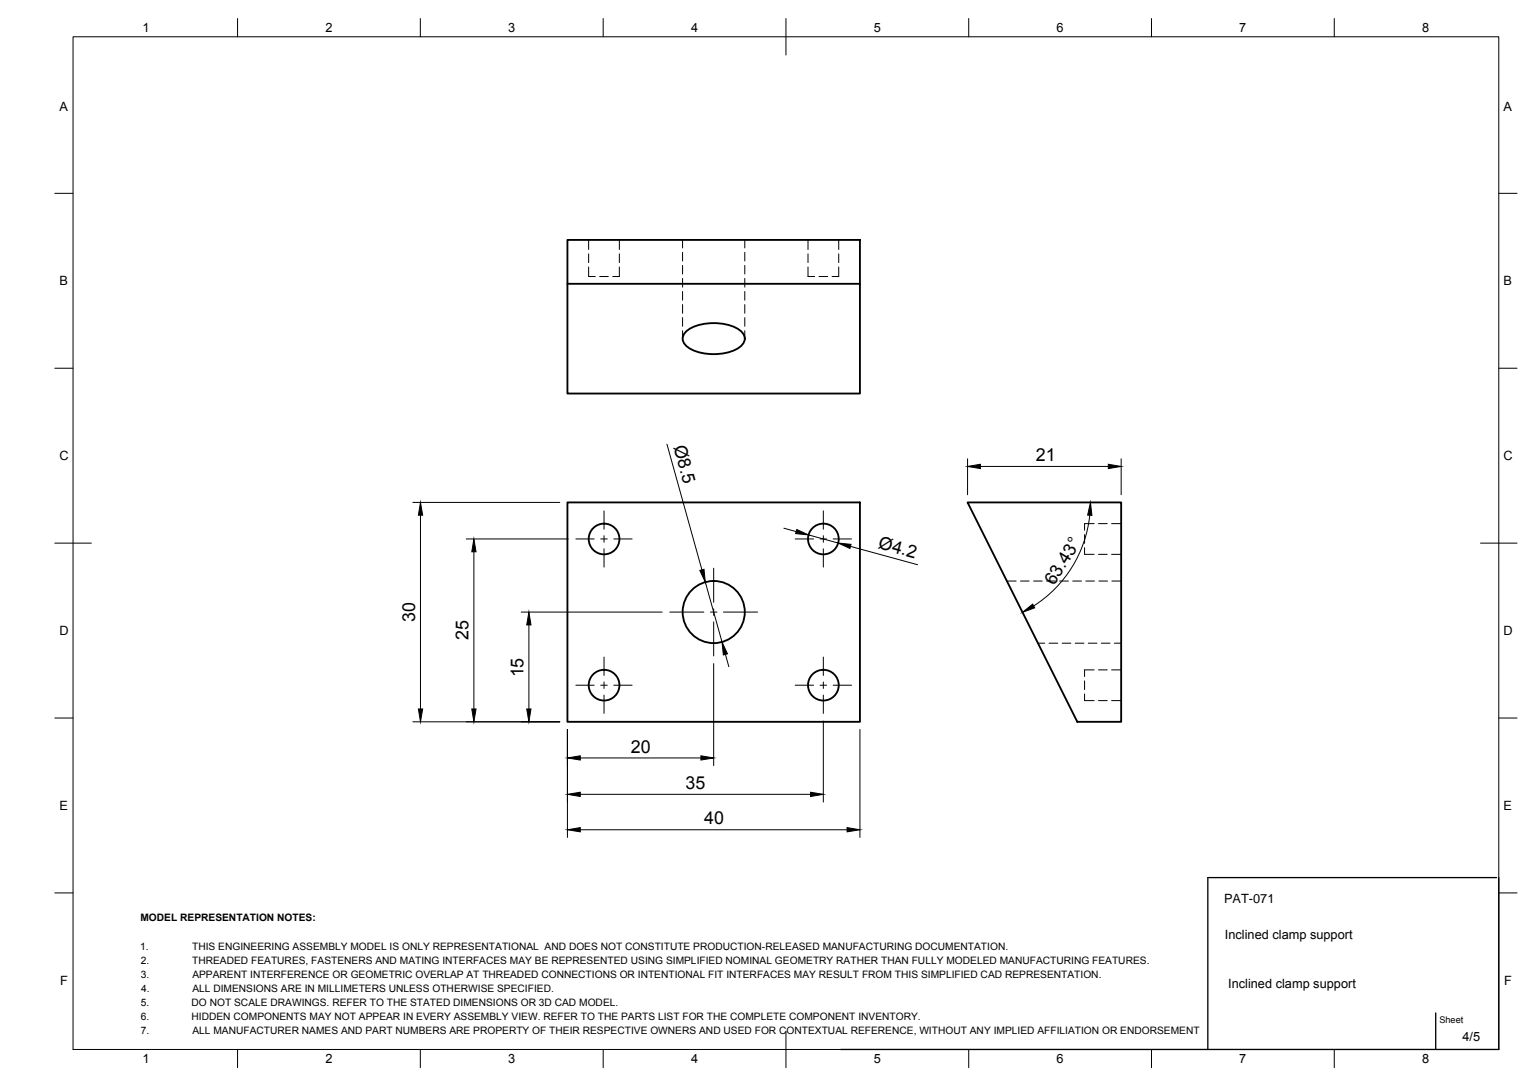
ISO-10303-21;
HEADER;
/* Generated by software containing ST-Developer
 * from STEP Tools, Inc. (www.steptools.com) 
 */

FILE_DESCRIPTION(
/* description */ ('Low-profile wedge edge clamp'),
/* implementation_level */ '2;1');

FILE_NAME(
/* name */ 'Inclined clamp support.step',
/* time_stamp */ '2026-10-29T15:58:13-07:00',
/* author */ (''),
/* organization */ (''),
/* preprocessor_version */ 'ST-DEVELOPER v20.2',
/* originating_system */ 'Autodesk Translation Framework v15.17.0.0',
/* authorisation */ '');

FILE_SCHEMA (('AUTOMOTIVE_DESIGN { 1 0 10303 214 3 1 1 }'));
ENDSEC;

DATA;
#10=MECHANICAL_DESIGN_GEOMETRIC_PRESENTATION_REPRESENTATION('',(#80),#2996);
#64=ELLIPSE('',#1900,0.475164445218705,0.425);
#68=SHAPE_REPRESENTATION_RELATIONSHIP('SRR','None',#3030,#74);
#74=ADVANCED_BREP_SHAPE_REPRESENTATION('',(#86),#2991);
#80=STYLED_ITEM('',(#3119),#86);
#86=MANIFOLD_SOLID_BREP('Body1',#1709);
#150=FACE_BOUND('',#408,.T.);
#151=FACE_BOUND('',#409,.T.);
#152=FACE_BOUND('',#410,.T.);
#153=FACE_BOUND('',#411,.T.);
#154=FACE_BOUND('',#412,.T.);
#155=FACE_BOUND('',#415,.T.);
#168=PLANE('',#1885);
#169=PLANE('',#1889);
#170=PLANE('',#1893);
#171=PLANE('',#1897);
#172=PLANE('',#1901);
#173=PLANE('',#1902);
#174=PLANE('',#1903);
#175=PLANE('',#1904);
#176=PLANE('',#1905);
#177=PLANE('',#1906);
#244=FACE_OUTER_BOUND('',#397,.T.);
#245=FACE_OUTER_BOUND('',#398,.T.);
#246=FACE_OUTER_BOUND('',#399,.T.);
#247=FACE_OUTER_BOUND('',#400,.T.);
#248=FACE_OUTER_BOUND('',#401,.T.);
#249=FACE_OUTER_BOUND('',#402,.T.);
#250=FACE_OUTER_BOUND('',#403,.T.);
#251=FACE_OUTER_BOUND('',#404,.T.);
#252=FACE_OUTER_BOUND('',#405,.T.);
#253=FACE_OUTER_BOUND('',#406,.T.);
#254=FACE_OUTER_BOUND('',#407,.T.);
#255=FACE_OUTER_BOUND('',#413,.T.);
#256=FACE_OUTER_BOUND('',#414,.T.);
#257=FACE_OUTER_BOUND('',#416,.T.);
#258=FACE_OUTER_BOUND('',#417,.T.);
#397=EDGE_LOOP('',(#1349,#1350,#1351,#1352));
#398=EDGE_LOOP('',(#1353));
#399=EDGE_LOOP('',(#1354,#1355,#1356,#1357));
#400=EDGE_LOOP('',(#1358));
#401=EDGE_LOOP('',(#1359,#1360,#1361,#1362));
#402=EDGE_LOOP('',(#1363));
#403=EDGE_LOOP('',(#1364,#1365,#1366,#1367));
#404=EDGE_LOOP('',(#1368));
#405=EDGE_LOOP('',(#1369,#1370,#1371,#1372));
#406=EDGE_LOOP('',(#1373,#1374,#1375,#1376));
#407=EDGE_LOOP('',(#1377,#1378,#1379,#1380));
#408=EDGE_LOOP('',(#1381));
#409=EDGE_LOOP('',(#1382));
#410=EDGE_LOOP('',(#1383));
#411=EDGE_LOOP('',(#1384));
#412=EDGE_LOOP('',(#1385));
#413=EDGE_LOOP('',(#1386,#1387,#1388,#1389));
#414=EDGE_LOOP('',(#1390,#1391,#1392,#1393));
#415=EDGE_LOOP('',(#1394));
#416=EDGE_LOOP('',(#1395,#1396,#1397,#1398));
#417=EDGE_LOOP('',(#1399,#1400,#1401,#1402));
#508=LINE('',#2715,#627);
#509=LINE('',#2722,#628);
#510=LINE('',#2729,#629);
#511=LINE('',#2736,#630);
#512=LINE('',#2743,#631);
#513=LINE('',#2748,#632);
#514=LINE('',#2750,#633);
#515=LINE('',#2752,#634);
#516=LINE('',#2753,#635);
#517=LINE('',#2756,#636);
#518=LINE('',#2758,#637);
#519=LINE('',#2759,#638);
#520=LINE('',#2762,#639);
#521=LINE('',#2764,#640);
#522=LINE('',#2765,#641);
#523=LINE('',#2767,#642);
#524=LINE('',#2768,#643);
#627=VECTOR('',#2228,0.21);
#628=VECTOR('',#2237,0.21);
#629=VECTOR('',#2246,0.21);
#630=VECTOR('',#2255,0.21);
#631=VECTOR('',#2264,0.425);
#632=VECTOR('',#2269,1.);
#633=VECTOR('',#2270,1.);
#634=VECTOR('',#2271,1.);
#635=VECTOR('',#2272,1.);
#636=VECTOR('',#2275,1.);
#637=VECTOR('',#2276,1.);
#638=VECTOR('',#2277,1.);
#639=VECTOR('',#2280,1.);
#640=VECTOR('',#2281,1.);
#641=VECTOR('',#2282,1.);
#642=VECTOR('',#2285,1.);
#643=VECTOR('',#2286,1.);
#764=CIRCLE('',#1883,0.21);
#765=CIRCLE('',#1884,0.21);
#766=CIRCLE('',#1887,0.21);
#767=CIRCLE('',#1888,0.21);
#768=CIRCLE('',#1891,0.21);
#769=CIRCLE('',#1892,0.21);
#770=CIRCLE('',#1895,0.21);
#771=CIRCLE('',#1896,0.21);
#772=CIRCLE('',#1899,0.425);
#858=VERTEX_POINT('',#2712);
#859=VERTEX_POINT('',#2714);
#860=VERTEX_POINT('',#2719);
#861=VERTEX_POINT('',#2721);
#862=VERTEX_POINT('',#2726);
#863=VERTEX_POINT('',#2728);
#864=VERTEX_POINT('',#2733);
#865=VERTEX_POINT('',#2735);
#866=VERTEX_POINT('',#2740);
#867=VERTEX_POINT('',#2742);
#868=VERTEX_POINT('',#2746);
#869=VERTEX_POINT('',#2747);
#870=VERTEX_POINT('',#2749);
#871=VERTEX_POINT('',#2751);
#872=VERTEX_POINT('',#2755);
#873=VERTEX_POINT('',#2757);
#874=VERTEX_POINT('',#2761);
#875=VERTEX_POINT('',#2763);
#1033=EDGE_CURVE('',#858,#858,#764,.T.);
#1034=EDGE_CURVE('',#858,#859,#508,.T.);
#1035=EDGE_CURVE('',#859,#859,#765,.T.);
#1036=EDGE_CURVE('',#860,#860,#766,.T.);
#1037=EDGE_CURVE('',#860,#861,#509,.T.);
#1038=EDGE_CURVE('',#861,#861,#767,.T.);
#1039=EDGE_CURVE('',#862,#862,#768,.T.);
#1040=EDGE_CURVE('',#862,#863,#510,.T.);
#1041=EDGE_CURVE('',#863,#863,#769,.T.);
#1042=EDGE_CURVE('',#864,#864,#770,.T.);
#1043=EDGE_CURVE('',#864,#865,#511,.T.);
#1044=EDGE_CURVE('',#865,#865,#771,.T.);
#1045=EDGE_CURVE('',#866,#866,#772,.T.);
#1046=EDGE_CURVE('',#866,#867,#512,.T.);
#1047=EDGE_CURVE('',#867,#867,#64,.T.);
#1048=EDGE_CURVE('',#868,#869,#513,.T.);
#1049=EDGE_CURVE('',#868,#870,#514,.T.);
#1050=EDGE_CURVE('',#871,#870,#515,.T.);
#1051=EDGE_CURVE('',#869,#871,#516,.T.);
#1052=EDGE_CURVE('',#869,#872,#517,.T.);
#1053=EDGE_CURVE('',#873,#871,#518,.T.);
#1054=EDGE_CURVE('',#872,#873,#519,.T.);
#1055=EDGE_CURVE('',#872,#874,#520,.T.);
#1056=EDGE_CURVE('',#875,#873,#521,.T.);
#1057=EDGE_CURVE('',#874,#875,#522,.T.);
#1058=EDGE_CURVE('',#874,#868,#523,.T.);
#1059=EDGE_CURVE('',#870,#875,#524,.T.);
#1349=ORIENTED_EDGE('',*,*,#1033,.F.);
#1350=ORIENTED_EDGE('',*,*,#1034,.T.);
#1351=ORIENTED_EDGE('',*,*,#1035,.T.);
#1352=ORIENTED_EDGE('',*,*,#1034,.F.);
#1353=ORIENTED_EDGE('',*,*,#1035,.F.);
#1354=ORIENTED_EDGE('',*,*,#1036,.F.);
#1355=ORIENTED_EDGE('',*,*,#1037,.T.);
#1356=ORIENTED_EDGE('',*,*,#1038,.T.);
#1357=ORIENTED_EDGE('',*,*,#1037,.F.);
#1358=ORIENTED_EDGE('',*,*,#1038,.F.);
#1359=ORIENTED_EDGE('',*,*,#1039,.F.);
#1360=ORIENTED_EDGE('',*,*,#1040,.T.);
#1361=ORIENTED_EDGE('',*,*,#1041,.T.);
#1362=ORIENTED_EDGE('',*,*,#1040,.F.);
#1363=ORIENTED_EDGE('',*,*,#1041,.F.);
#1364=ORIENTED_EDGE('',*,*,#1042,.F.);
#1365=ORIENTED_EDGE('',*,*,#1043,.T.);
#1366=ORIENTED_EDGE('',*,*,#1044,.T.);
#1367=ORIENTED_EDGE('',*,*,#1043,.F.);
#1368=ORIENTED_EDGE('',*,*,#1044,.F.);
#1369=ORIENTED_EDGE('',*,*,#1045,.F.);
#1370=ORIENTED_EDGE('',*,*,#1046,.T.);
#1371=ORIENTED_EDGE('',*,*,#1047,.F.);
#1372=ORIENTED_EDGE('',*,*,#1046,.F.);
#1373=ORIENTED_EDGE('',*,*,#1048,.F.);
#1374=ORIENTED_EDGE('',*,*,#1049,.T.);
#1375=ORIENTED_EDGE('',*,*,#1050,.F.);
#1376=ORIENTED_EDGE('',*,*,#1051,.F.);
#1377=ORIENTED_EDGE('',*,*,#1052,.F.);
#1378=ORIENTED_EDGE('',*,*,#1051,.T.);
#1379=ORIENTED_EDGE('',*,*,#1053,.F.);
#1380=ORIENTED_EDGE('',*,*,#1054,.F.);
#1381=ORIENTED_EDGE('',*,*,#1045,.T.);
#1382=ORIENTED_EDGE('',*,*,#1042,.T.);
#1383=ORIENTED_EDGE('',*,*,#1039,.T.);
#1384=ORIENTED_EDGE('',*,*,#1036,.T.);
#1385=ORIENTED_EDGE('',*,*,#1033,.T.);
#1386=ORIENTED_EDGE('',*,*,#1055,.F.);
#1387=ORIENTED_EDGE('',*,*,#1054,.T.);
#1388=ORIENTED_EDGE('',*,*,#1056,.F.);
#1389=ORIENTED_EDGE('',*,*,#1057,.F.);
#1390=ORIENTED_EDGE('',*,*,#1058,.F.);
#1391=ORIENTED_EDGE('',*,*,#1057,.T.);
#1392=ORIENTED_EDGE('',*,*,#1059,.F.);
#1393=ORIENTED_EDGE('',*,*,#1049,.F.);
#1394=ORIENTED_EDGE('',*,*,#1047,.T.);
#1395=ORIENTED_EDGE('',*,*,#1059,.T.);
#1396=ORIENTED_EDGE('',*,*,#1056,.T.);
#1397=ORIENTED_EDGE('',*,*,#1053,.T.);
#1398=ORIENTED_EDGE('',*,*,#1050,.T.);
#1399=ORIENTED_EDGE('',*,*,#1058,.T.);
#1400=ORIENTED_EDGE('',*,*,#1048,.T.);
#1401=ORIENTED_EDGE('',*,*,#1052,.T.);
#1402=ORIENTED_EDGE('',*,*,#1055,.T.);
#1603=CYLINDRICAL_SURFACE('',#1882,0.21);
#1604=CYLINDRICAL_SURFACE('',#1886,0.21);
#1605=CYLINDRICAL_SURFACE('',#1890,0.21);
#1606=CYLINDRICAL_SURFACE('',#1894,0.21);
#1607=CYLINDRICAL_SURFACE('',#1898,0.425);
#1651=ADVANCED_FACE('',(#244),#1603,.F.);
#1652=ADVANCED_FACE('',(#245),#168,.F.);
#1653=ADVANCED_FACE('',(#246),#1604,.F.);
#1654=ADVANCED_FACE('',(#247),#169,.F.);
#1655=ADVANCED_FACE('',(#248),#1605,.F.);
#1656=ADVANCED_FACE('',(#249),#170,.F.);
#1657=ADVANCED_FACE('',(#250),#1606,.F.);
#1658=ADVANCED_FACE('',(#251),#171,.F.);
#1659=ADVANCED_FACE('',(#252),#1607,.F.);
#1660=ADVANCED_FACE('',(#253),#172,.T.);
#1661=ADVANCED_FACE('',(#254,#150,#151,#152,#153,#154),#173,.T.);
#1662=ADVANCED_FACE('',(#255),#174,.T.);
#1663=ADVANCED_FACE('',(#256,#155),#175,.T.);
#1664=ADVANCED_FACE('',(#257),#176,.T.);
#1665=ADVANCED_FACE('',(#258),#177,.F.);
#1709=CLOSED_SHELL('',(#1651,#1652,#1653,#1654,#1655,#1656,#1657,#1658,
#1659,#1660,#1661,#1662,#1663,#1664,#1665));
#1881=AXIS2_PLACEMENT_3D('',#2710,#2222,#2223);
#1882=AXIS2_PLACEMENT_3D('',#2711,#2224,#2225);
#1883=AXIS2_PLACEMENT_3D('',#2713,#2226,#2227);
#1884=AXIS2_PLACEMENT_3D('',#2716,#2229,#2230);
#1885=AXIS2_PLACEMENT_3D('',#2717,#2231,#2232);
#1886=AXIS2_PLACEMENT_3D('',#2718,#2233,#2234);
#1887=AXIS2_PLACEMENT_3D('',#2720,#2235,#2236);
#1888=AXIS2_PLACEMENT_3D('',#2723,#2238,#2239);
#1889=AXIS2_PLACEMENT_3D('',#2724,#2240,#2241);
#1890=AXIS2_PLACEMENT_3D('',#2725,#2242,#2243);
#1891=AXIS2_PLACEMENT_3D('',#2727,#2244,#2245);
#1892=AXIS2_PLACEMENT_3D('',#2730,#2247,#2248);
#1893=AXIS2_PLACEMENT_3D('',#2731,#2249,#2250);
#1894=AXIS2_PLACEMENT_3D('',#2732,#2251,#2252);
#1895=AXIS2_PLACEMENT_3D('',#2734,#2253,#2254);
#1896=AXIS2_PLACEMENT_3D('',#2737,#2256,#2257);
#1897=AXIS2_PLACEMENT_3D('',#2738,#2258,#2259);
#1898=AXIS2_PLACEMENT_3D('',#2739,#2260,#2261);
#1899=AXIS2_PLACEMENT_3D('',#2741,#2262,#2263);
#1900=AXIS2_PLACEMENT_3D('',#2744,#2265,#2266);
#1901=AXIS2_PLACEMENT_3D('',#2745,#2267,#2268);
#1902=AXIS2_PLACEMENT_3D('',#2754,#2273,#2274);
#1903=AXIS2_PLACEMENT_3D('',#2760,#2278,#2279);
#1904=AXIS2_PLACEMENT_3D('',#2766,#2283,#2284);
#1905=AXIS2_PLACEMENT_3D('',#2769,#2287,#2288);
#1906=AXIS2_PLACEMENT_3D('',#2770,#2289,#2290);
#2222=DIRECTION('axis',(0.,0.,1.));
#2223=DIRECTION('refdir',(1.,0.,0.));
#2224=DIRECTION('center_axis',(0.,0.,1.));
#2225=DIRECTION('ref_axis',(1.,0.,0.));
#2226=DIRECTION('center_axis',(0.,0.,1.));
#2227=DIRECTION('ref_axis',(1.,0.,0.));
#2228=DIRECTION('',(0.,0.,1.));
#2229=DIRECTION('center_axis',(0.,0.,1.));
#2230=DIRECTION('ref_axis',(1.,0.,0.));
#2231=DIRECTION('center_axis',(0.,0.,1.));
#2232=DIRECTION('ref_axis',(1.,0.,0.));
#2233=DIRECTION('center_axis',(0.,0.,1.));
#2234=DIRECTION('ref_axis',(1.,0.,0.));
#2235=DIRECTION('center_axis',(0.,0.,1.));
#2236=DIRECTION('ref_axis',(1.,0.,0.));
#2237=DIRECTION('',(0.,0.,1.));
#2238=DIRECTION('center_axis',(0.,0.,1.));
#2239=DIRECTION('ref_axis',(1.,0.,0.));
#2240=DIRECTION('center_axis',(0.,0.,1.));
#2241=DIRECTION('ref_axis',(1.,0.,0.));
#2242=DIRECTION('center_axis',(0.,0.,1.));
#2243=DIRECTION('ref_axis',(1.,0.,0.));
#2244=DIRECTION('center_axis',(0.,0.,1.));
#2245=DIRECTION('ref_axis',(1.,0.,0.));
#2246=DIRECTION('',(0.,0.,1.));
#2247=DIRECTION('center_axis',(0.,0.,1.));
#2248=DIRECTION('ref_axis',(1.,0.,0.));
#2249=DIRECTION('center_axis',(0.,0.,1.));
#2250=DIRECTION('ref_axis',(1.,0.,0.));
#2251=DIRECTION('center_axis',(0.,0.,1.));
#2252=DIRECTION('ref_axis',(1.,0.,0.));
#2253=DIRECTION('center_axis',(0.,0.,1.));
#2254=DIRECTION('ref_axis',(1.,0.,0.));
#2255=DIRECTION('',(0.,0.,1.));
#2256=DIRECTION('center_axis',(0.,0.,1.));
#2257=DIRECTION('ref_axis',(1.,0.,0.));
#2258=DIRECTION('center_axis',(0.,0.,1.));
#2259=DIRECTION('ref_axis',(1.,0.,0.));
#2260=DIRECTION('center_axis',(0.,0.,1.));
#2261=DIRECTION('ref_axis',(1.,0.,0.));
#2262=DIRECTION('center_axis',(0.,0.,1.));
#2263=DIRECTION('ref_axis',(1.,0.,0.));
#2264=DIRECTION('',(0.,0.,1.));
#2265=DIRECTION('center_axis',(0.447213595499958,0.,-0.894427190999916));
#2266=DIRECTION('ref_axis',(0.894427190999916,0.,0.447213595499958));
#2267=DIRECTION('center_axis',(-1.,0.,0.));
#2268=DIRECTION('ref_axis',(0.,0.,1.));
#2269=DIRECTION('',(0.,0.,-1.));
#2270=DIRECTION('',(0.,1.,0.));
#2271=DIRECTION('',(0.,0.,1.));
#2272=DIRECTION('',(0.,1.,0.));
#2273=DIRECTION('center_axis',(0.,0.,-1.));
#2274=DIRECTION('ref_axis',(-1.,0.,0.));
#2275=DIRECTION('',(1.,0.,0.));
#2276=DIRECTION('',(-1.,0.,0.));
#2277=DIRECTION('',(0.,1.,0.));
#2278=DIRECTION('center_axis',(1.,0.,0.));
#2279=DIRECTION('ref_axis',(0.,0.,-1.));
#2280=DIRECTION('',(0.,0.,1.));
#2281=DIRECTION('',(0.,0.,-1.));
#2282=DIRECTION('',(0.,1.,0.));
#2283=DIRECTION('center_axis',(-0.447213595499958,0.,0.894427190999916));
#2284=DIRECTION('ref_axis',(0.894427190999916,0.,0.447213595499958));
#2285=DIRECTION('',(-0.894427190999916,0.,-0.447213595499958));
#2286=DIRECTION('',(0.894427190999916,0.,0.447213595499958));
#2287=DIRECTION('center_axis',(0.,1.,0.));
#2288=DIRECTION('ref_axis',(0.,0.,1.));
#2289=DIRECTION('center_axis',(0.,1.,0.));
#2290=DIRECTION('ref_axis',(1.,0.,0.));
#2710=CARTESIAN_POINT('',(0.,0.,0.));
#2711=CARTESIAN_POINT('Origin',(2.5,-1.5,0.9));
#2712=CARTESIAN_POINT('',(2.29,-1.5,1.));
#2713=CARTESIAN_POINT('Origin',(2.5,-1.5,1.));
#2714=CARTESIAN_POINT('',(2.29,-1.5,1.5));
#2715=CARTESIAN_POINT('',(2.29,-1.5,0.9));
#2716=CARTESIAN_POINT('Origin',(2.5,-1.5,1.5));
#2717=CARTESIAN_POINT('Origin',(2.5,-1.5,1.5));
#2718=CARTESIAN_POINT('Origin',(0.5,1.5,0.9));
#2719=CARTESIAN_POINT('',(0.29,1.5,1.));
#2720=CARTESIAN_POINT('Origin',(0.5,1.5,1.));
#2721=CARTESIAN_POINT('',(0.29,1.5,1.5));
#2722=CARTESIAN_POINT('',(0.29,1.5,0.9));
#2723=CARTESIAN_POINT('Origin',(0.5,1.5,1.5));
#2724=CARTESIAN_POINT('Origin',(0.5,1.5,1.5));
#2725=CARTESIAN_POINT('Origin',(0.5,-1.5,0.9));
#2726=CARTESIAN_POINT('',(0.29,-1.5,1.));
#2727=CARTESIAN_POINT('Origin',(0.5,-1.5,1.));
#2728=CARTESIAN_POINT('',(0.29,-1.5,1.5));
#2729=CARTESIAN_POINT('',(0.29,-1.5,0.9));
#2730=CARTESIAN_POINT('Origin',(0.5,-1.5,1.5));
#2731=CARTESIAN_POINT('Origin',(0.5,-1.5,1.5));
#2732=CARTESIAN_POINT('Origin',(2.5,1.5,0.9));
#2733=CARTESIAN_POINT('',(2.29,1.5,1.));
#2734=CARTESIAN_POINT('Origin',(2.5,1.5,1.));
#2735=CARTESIAN_POINT('',(2.29,1.5,1.5));
#2736=CARTESIAN_POINT('',(2.29,1.5,0.9));
#2737=CARTESIAN_POINT('Origin',(2.5,1.5,1.5));
#2738=CARTESIAN_POINT('Origin',(2.5,1.5,1.5));
#2739=CARTESIAN_POINT('Origin',(1.5,0.,0.9));
#2740=CARTESIAN_POINT('',(1.075,-5.20474889637625E-17,1.));
#2741=CARTESIAN_POINT('Origin',(1.5,0.,1.));
#2742=CARTESIAN_POINT('',(1.075,5.20474889637625E-17,2.1375));
#2743=CARTESIAN_POINT('',(1.075,-5.20474889637625E-17,0.9));
#2744=CARTESIAN_POINT('Origin',(1.5,0.,2.35));
#2745=CARTESIAN_POINT('Origin',(0.,-2.,1.));
#2746=CARTESIAN_POINT('',(0.,-2.,1.6));
#2747=CARTESIAN_POINT('',(0.,-2.,1.));
#2748=CARTESIAN_POINT('',(0.,-2.,1.6));
#2749=CARTESIAN_POINT('',(0.,2.,1.6));
#2750=CARTESIAN_POINT('',(0.,-2.,1.6));
#2751=CARTESIAN_POINT('',(0.,2.,1.));
#2752=CARTESIAN_POINT('',(0.,2.,1.6));
#2753=CARTESIAN_POINT('',(0.,-2.,1.));
#2754=CARTESIAN_POINT('Origin',(3.,-2.,1.));
#2755=CARTESIAN_POINT('',(3.,-2.,1.));
#2756=CARTESIAN_POINT('',(0.,-2.,1.));
#2757=CARTESIAN_POINT('',(3.,2.,1.));
#2758=CARTESIAN_POINT('',(0.,2.,1.));
#2759=CARTESIAN_POINT('',(3.,-2.,1.));
#2760=CARTESIAN_POINT('Origin',(3.,-2.,3.1));
#2761=CARTESIAN_POINT('',(3.,-2.,3.1));
#2762=CARTESIAN_POINT('',(3.,-2.,1.));
#2763=CARTESIAN_POINT('',(3.,2.,3.1));
#2764=CARTESIAN_POINT('',(3.,2.,1.));
#2765=CARTESIAN_POINT('',(3.,-2.,3.1));
#2766=CARTESIAN_POINT('Origin',(0.,-2.,1.6));
#2767=CARTESIAN_POINT('',(3.,-2.,3.1));
#2768=CARTESIAN_POINT('',(3.,2.,3.1));
#2769=CARTESIAN_POINT('Origin',(1.5,2.,2.05));
#2770=CARTESIAN_POINT('Origin',(1.5,-2.,2.05));
#2982=UNCERTAINTY_MEASURE_WITH_UNIT(LENGTH_MEASURE(0.001),#2997,
'DISTANCE_ACCURACY_VALUE',
'Maximum model space distance between geometric entities at asserted c
onnectivities');
#2987=UNCERTAINTY_MEASURE_WITH_UNIT(LENGTH_MEASURE(0.001),#2997,
'DISTANCE_ACCURACY_VALUE',
'Maximum model space distance between geometric entities at asserted c
onnectivities');
#2991=(
GEOMETRIC_REPRESENTATION_CONTEXT(3)
GLOBAL_UNCERTAINTY_ASSIGNED_CONTEXT((#2982))
GLOBAL_UNIT_ASSIGNED_CONTEXT((#2997,#2999,#3000))
REPRESENTATION_CONTEXT('','3D')
);
#2996=(
GEOMETRIC_REPRESENTATION_CONTEXT(3)
GLOBAL_UNCERTAINTY_ASSIGNED_CONTEXT((#2987))
GLOBAL_UNIT_ASSIGNED_CONTEXT((#2997,#2999,#3000))
REPRESENTATION_CONTEXT('','3D')
);
#2997=(
LENGTH_UNIT()
NAMED_UNIT(*)
SI_UNIT(.CENTI.,.METRE.)
);
#2999=(
NAMED_UNIT(*)
PLANE_ANGLE_UNIT()
SI_UNIT($,.RADIAN.)
);
#3000=(
NAMED_UNIT(*)
SI_UNIT($,.STERADIAN.)
SOLID_ANGLE_UNIT()
);
#3004=SHAPE_DEFINITION_REPRESENTATION(#3012,#3030);
#3012=PRODUCT_DEFINITION_SHAPE('',$,#3039);
#3030=SHAPE_REPRESENTATION('',(#1881),#2991);
#3035=PRODUCT_DEFINITION_CONTEXT('part definition',#3061,'design');
#3039=PRODUCT_DEFINITION('Inclined clamp support',
'Inclined clamp support',#3047,#3035);
#3047=PRODUCT_DEFINITION_FORMATION('',$,#3066);
#3061=APPLICATION_CONTEXT(
'Core Data for Automotive Mechanical Design Process');
#3062=PRODUCT_CONTEXT('part definition',#3061,'mechanical');
#3066=PRODUCT('Inclined clamp support','Inclined clamp support',
'Inclined clamp support',(#3062));
#3113=COLOUR_RGB('Sky Blue',0.24,0.69,0.87);
#3114=FILL_AREA_STYLE_COLOUR('',#3113);
#3115=FILL_AREA_STYLE('',(#3114));
#3116=SURFACE_STYLE_FILL_AREA(#3115);
#3117=SURFACE_SIDE_STYLE('',(#3116));
#3118=SURFACE_STYLE_USAGE(.BOTH.,#3117);
#3119=PRESENTATION_STYLE_ASSIGNMENT((#3118));
ENDSEC;
END-ISO-10303-21;
